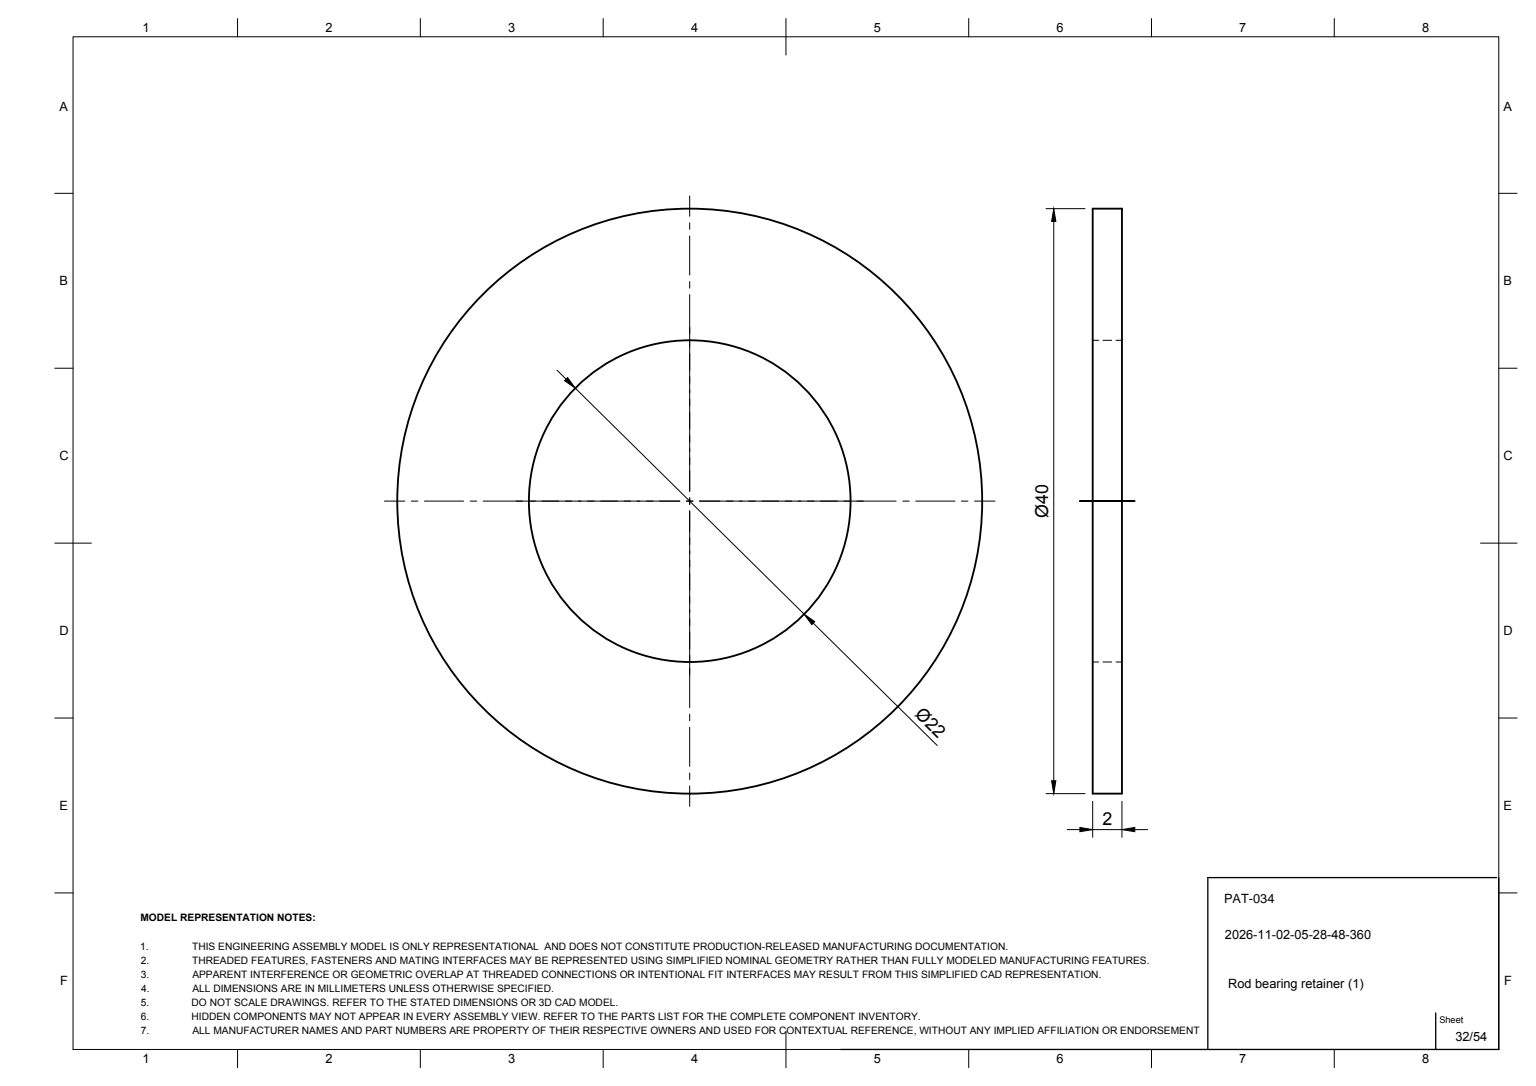
ISO-10303-21;
HEADER;
/* Generated by software containing ST-Developer
 * from STEP Tools, Inc. (www.steptools.com) 
 */

FILE_DESCRIPTION(
/* description */ ('Fatigue rig crank-slider'),
/* implementation_level */ '2;1');

FILE_NAME(
/* name */ 'Rod bearing retainer (1).step',
/* time_stamp */ '2026-10-28T03:24:50-07:00',
/* author */ (''),
/* organization */ (''),
/* preprocessor_version */ 'ST-DEVELOPER v20.2',
/* originating_system */ 'Autodesk Translation Framework v15.17.0.0',
/* authorisation */ '');

FILE_SCHEMA (('AUTOMOTIVE_DESIGN { 1 0 10303 214 3 1 1 }'));
ENDSEC;

DATA;
#10=MECHANICAL_DESIGN_GEOMETRIC_PRESENTATION_REPRESENTATION('',(#617),#16911);
#516=SHAPE_REPRESENTATION_RELATIONSHIP('SRR','None',#17158,#566);
#566=ADVANCED_BREP_SHAPE_REPRESENTATION('',(#674),#16887);
#617=STYLED_ITEM('',(#17487),#674);
#674=MANIFOLD_SOLID_BREP('Body1',#8910);
#848=FACE_BOUND('',#2204,.T.);
#849=FACE_BOUND('',#2206,.T.);
#1088=PLANE('',#10086);
#1089=PLANE('',#10087);
#1530=FACE_OUTER_BOUND('',#2201,.T.);
#1531=FACE_OUTER_BOUND('',#2202,.T.);
#1532=FACE_OUTER_BOUND('',#2203,.T.);
#1533=FACE_OUTER_BOUND('',#2205,.T.);
#2201=EDGE_LOOP('',(#7304,#7305,#7306,#7307));
#2202=EDGE_LOOP('',(#7308,#7309,#7310,#7311));
#2203=EDGE_LOOP('',(#7312));
#2204=EDGE_LOOP('',(#7313));
#2205=EDGE_LOOP('',(#7314));
#2206=EDGE_LOOP('',(#7315));
#2841=LINE('',#15388,#3487);
#2842=LINE('',#15394,#3488);
#3487=VECTOR('',#12125,1.1);
#3488=VECTOR('',#12132,2.);
#3989=CIRCLE('',#10081,1.1);
#3990=CIRCLE('',#10082,1.1);
#3991=CIRCLE('',#10084,2.);
#3992=CIRCLE('',#10085,2.);
#4593=VERTEX_POINT('',#15385);
#4594=VERTEX_POINT('',#15387);
#4595=VERTEX_POINT('',#15391);
#4596=VERTEX_POINT('',#15393);
#5550=EDGE_CURVE('',#4593,#4593,#3989,.T.);
#5551=EDGE_CURVE('',#4593,#4594,#2841,.T.);
#5552=EDGE_CURVE('',#4594,#4594,#3990,.T.);
#5553=EDGE_CURVE('',#4595,#4595,#3991,.T.);
#5554=EDGE_CURVE('',#4595,#4596,#2842,.T.);
#5555=EDGE_CURVE('',#4596,#4596,#3992,.T.);
#7304=ORIENTED_EDGE('',*,*,#5550,.F.);
#7305=ORIENTED_EDGE('',*,*,#5551,.T.);
#7306=ORIENTED_EDGE('',*,*,#5552,.T.);
#7307=ORIENTED_EDGE('',*,*,#5551,.F.);
#7308=ORIENTED_EDGE('',*,*,#5553,.F.);
#7309=ORIENTED_EDGE('',*,*,#5554,.T.);
#7310=ORIENTED_EDGE('',*,*,#5555,.T.);
#7311=ORIENTED_EDGE('',*,*,#5554,.F.);
#7312=ORIENTED_EDGE('',*,*,#5553,.T.);
#7313=ORIENTED_EDGE('',*,*,#5550,.T.);
#7314=ORIENTED_EDGE('',*,*,#5555,.F.);
#7315=ORIENTED_EDGE('',*,*,#5552,.F.);
#8307=CYLINDRICAL_SURFACE('',#10080,1.1);
#8308=CYLINDRICAL_SURFACE('',#10083,2.);
#8668=ADVANCED_FACE('',(#1530),#8307,.F.);
#8669=ADVANCED_FACE('',(#1531),#8308,.T.);
#8670=ADVANCED_FACE('',(#1532,#848),#1088,.T.);
#8671=ADVANCED_FACE('',(#1533,#849),#1089,.F.);
#8910=CLOSED_SHELL('',(#8668,#8669,#8670,#8671));
#10079=AXIS2_PLACEMENT_3D('',#15383,#12119,#12120);
#10080=AXIS2_PLACEMENT_3D('',#15384,#12121,#12122);
#10081=AXIS2_PLACEMENT_3D('',#15386,#12123,#12124);
#10082=AXIS2_PLACEMENT_3D('',#15389,#12126,#12127);
#10083=AXIS2_PLACEMENT_3D('',#15390,#12128,#12129);
#10084=AXIS2_PLACEMENT_3D('',#15392,#12130,#12131);
#10085=AXIS2_PLACEMENT_3D('',#15395,#12133,#12134);
#10086=AXIS2_PLACEMENT_3D('',#15396,#12135,#12136);
#10087=AXIS2_PLACEMENT_3D('',#15397,#12137,#12138);
#12119=DIRECTION('axis',(0.,0.,1.));
#12120=DIRECTION('refdir',(1.,0.,0.));
#12121=DIRECTION('center_axis',(0.,1.,0.));
#12122=DIRECTION('ref_axis',(1.,0.,0.));
#12123=DIRECTION('center_axis',(0.,-1.,0.));
#12124=DIRECTION('ref_axis',(1.,0.,0.));
#12125=DIRECTION('',(0.,-1.,0.));
#12126=DIRECTION('center_axis',(0.,-1.,0.));
#12127=DIRECTION('ref_axis',(1.,0.,0.));
#12128=DIRECTION('center_axis',(0.,1.,0.));
#12129=DIRECTION('ref_axis',(1.,0.,0.));
#12130=DIRECTION('center_axis',(0.,1.,0.));
#12131=DIRECTION('ref_axis',(1.,0.,0.));
#12132=DIRECTION('',(0.,-1.,0.));
#12133=DIRECTION('center_axis',(0.,1.,0.));
#12134=DIRECTION('ref_axis',(1.,0.,0.));
#12135=DIRECTION('center_axis',(0.,1.,0.));
#12136=DIRECTION('ref_axis',(1.,0.,0.));
#12137=DIRECTION('center_axis',(0.,1.,0.));
#12138=DIRECTION('ref_axis',(1.,0.,0.));
#15383=CARTESIAN_POINT('',(0.,0.,0.));
#15384=CARTESIAN_POINT('Origin',(1.,4.4,12.));
#15385=CARTESIAN_POINT('',(-0.1,4.6,12.));
#15386=CARTESIAN_POINT('Origin',(1.,4.6,12.));
#15387=CARTESIAN_POINT('',(-0.1,4.4,12.));
#15388=CARTESIAN_POINT('',(-0.1,4.4,12.));
#15389=CARTESIAN_POINT('Origin',(1.,4.4,12.));
#15390=CARTESIAN_POINT('Origin',(1.,4.4,12.));
#15391=CARTESIAN_POINT('',(-1.,4.6,12.));
#15392=CARTESIAN_POINT('Origin',(1.,4.6,12.));
#15393=CARTESIAN_POINT('',(-1.,4.4,12.));
#15394=CARTESIAN_POINT('',(-1.,4.4,12.));
#15395=CARTESIAN_POINT('Origin',(1.,4.4,12.));
#15396=CARTESIAN_POINT('Origin',(1.,4.6,12.));
#15397=CARTESIAN_POINT('Origin',(1.,4.4,12.));
#16828=UNCERTAINTY_MEASURE_WITH_UNIT(LENGTH_MEASURE(0.001),#16912,
'DISTANCE_ACCURACY_VALUE',
'Maximum model space distance between geometric entities at asserted c
onnectivities');
#16852=UNCERTAINTY_MEASURE_WITH_UNIT(LENGTH_MEASURE(0.001),#16912,
'DISTANCE_ACCURACY_VALUE',
'Maximum model space distance between geometric entities at asserted c
onnectivities');
#16887=(
GEOMETRIC_REPRESENTATION_CONTEXT(3)
GLOBAL_UNCERTAINTY_ASSIGNED_CONTEXT((#16828))
GLOBAL_UNIT_ASSIGNED_CONTEXT((#16912,#16914,#16915))
REPRESENTATION_CONTEXT('','3D')
);
#16911=(
GEOMETRIC_REPRESENTATION_CONTEXT(3)
GLOBAL_UNCERTAINTY_ASSIGNED_CONTEXT((#16852))
GLOBAL_UNIT_ASSIGNED_CONTEXT((#16912,#16914,#16915))
REPRESENTATION_CONTEXT('','3D')
);
#16912=(
LENGTH_UNIT()
NAMED_UNIT(*)
SI_UNIT(.CENTI.,.METRE.)
);
#16914=(
NAMED_UNIT(*)
PLANE_ANGLE_UNIT()
SI_UNIT($,.RADIAN.)
);
#16915=(
NAMED_UNIT(*)
SI_UNIT($,.STERADIAN.)
SOLID_ANGLE_UNIT()
);
#16950=SHAPE_DEFINITION_REPRESENTATION(#17010,#17158);
#17010=PRODUCT_DEFINITION_SHAPE('',$,#17217);
#17158=SHAPE_REPRESENTATION('',(#10079),#16887);
#17182=PRODUCT_DEFINITION_CONTEXT('part definition',#17358,'design');
#17217=PRODUCT_DEFINITION('Rod bearing retainer (1)',
'Rod bearing retainer (1)',#17275,#17182);
#17275=PRODUCT_DEFINITION_FORMATION('',$,#17394);
#17358=APPLICATION_CONTEXT(
'Core Data for Automotive Mechanical Design Process');
#17359=PRODUCT_CONTEXT('part definition',#17358,'mechanical');
#17394=PRODUCT('Rod bearing retainer (1)','Rod bearing retainer (1)',
'Rod bearing retainer (1)',(#17359));
#17481=COLOUR_RGB('Grey',0.48,0.52,0.57);
#17482=FILL_AREA_STYLE_COLOUR('',#17481);
#17483=FILL_AREA_STYLE('',(#17482));
#17484=SURFACE_STYLE_FILL_AREA(#17483);
#17485=SURFACE_SIDE_STYLE('',(#17484));
#17486=SURFACE_STYLE_USAGE(.BOTH.,#17485);
#17487=PRESENTATION_STYLE_ASSIGNMENT((#17486));
ENDSEC;
END-ISO-10303-21;
